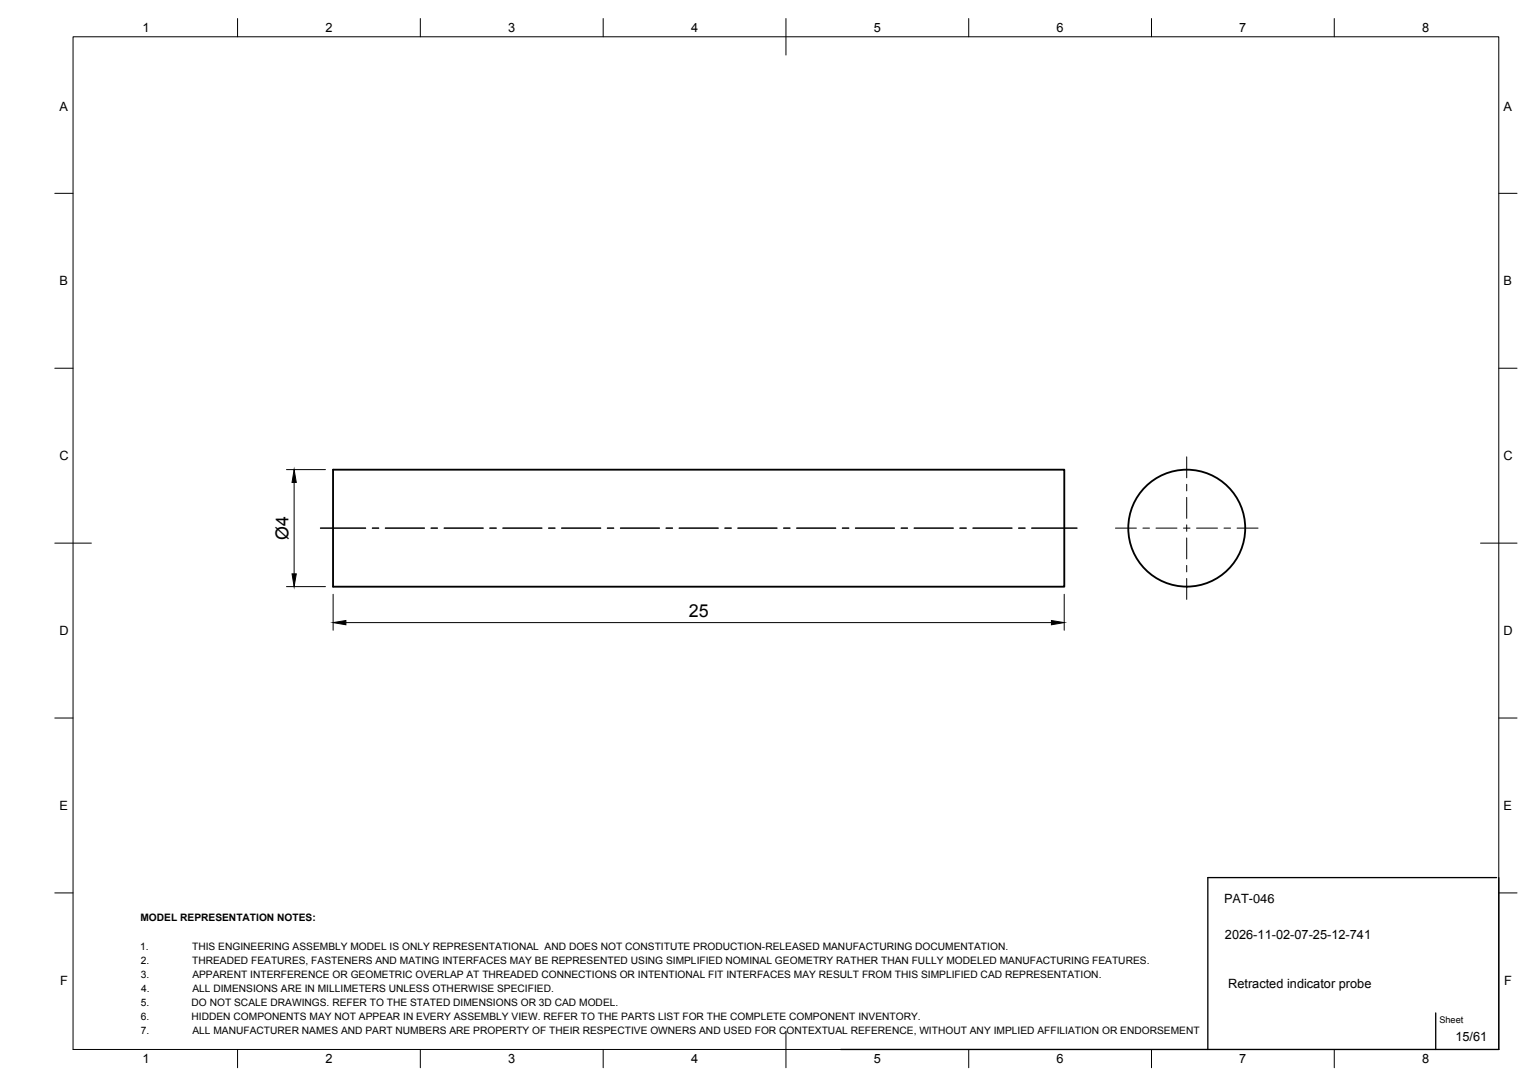
ISO-10303-21;
HEADER;
/* Generated by software containing ST-Developer
 * from STEP Tools, Inc. (www.steptools.com) 
 */

FILE_DESCRIPTION(
/* description */ ('Gear mesh backlash fixture'),
/* implementation_level */ '2;1');

FILE_NAME(
/* name */ 'Retracted indicator probe.step',
/* time_stamp */ '2026-10-28T03:26:00-07:00',
/* author */ (''),
/* organization */ (''),
/* preprocessor_version */ 'ST-DEVELOPER v20.2',
/* originating_system */ 'Autodesk Translation Framework v15.17.0.0',
/* authorisation */ '');

FILE_SCHEMA (('AUTOMOTIVE_DESIGN { 1 0 10303 214 3 1 1 }'));
ENDSEC;

DATA;
#10=MECHANICAL_DESIGN_GEOMETRIC_PRESENTATION_REPRESENTATION('',(#1026),#57900);
#926=SHAPE_REPRESENTATION_RELATIONSHIP('SRR','None',#58121,#976);
#976=ADVANCED_BREP_SHAPE_REPRESENTATION('',(#1091),#57854);
#1026=STYLED_ITEM('',(#58458),#1091);
#1091=MANIFOLD_SOLID_BREP('Body1',#13586);
#1393=PLANE('',#14451);
#1394=PLANE('',#14452);
#1811=FACE_OUTER_BOUND('',#2638,.T.);
#1812=FACE_OUTER_BOUND('',#2639,.T.);
#1813=FACE_OUTER_BOUND('',#2640,.T.);
#2638=EDGE_LOOP('',(#9421,#9422,#9423,#9424));
#2639=EDGE_LOOP('',(#9425));
#2640=EDGE_LOOP('',(#9426));
#3552=LINE('',#19909,#4441);
#4441=VECTOR('',#16229,0.2);
#5312=CIRCLE('',#14449,0.2);
#5313=CIRCLE('',#14450,0.2);
#5957=VERTEX_POINT('',#19906);
#5958=VERTEX_POINT('',#19908);
#7297=EDGE_CURVE('',#5957,#5957,#5312,.T.);
#7298=EDGE_CURVE('',#5957,#5958,#3552,.T.);
#7299=EDGE_CURVE('',#5958,#5958,#5313,.T.);
#9421=ORIENTED_EDGE('',*,*,#7297,.F.);
#9422=ORIENTED_EDGE('',*,*,#7298,.T.);
#9423=ORIENTED_EDGE('',*,*,#7299,.T.);
#9424=ORIENTED_EDGE('',*,*,#7298,.F.);
#9425=ORIENTED_EDGE('',*,*,#7297,.T.);
#9426=ORIENTED_EDGE('',*,*,#7299,.F.);
#12639=CYLINDRICAL_SURFACE('',#14448,0.2);
#12928=ADVANCED_FACE('',(#1811),#12639,.T.);
#12929=ADVANCED_FACE('',(#1812),#1393,.T.);
#12930=ADVANCED_FACE('',(#1813),#1394,.F.);
#13586=CLOSED_SHELL('',(#12928,#12929,#12930));
#14447=AXIS2_PLACEMENT_3D('',#19904,#16223,#16224);
#14448=AXIS2_PLACEMENT_3D('',#19905,#16225,#16226);
#14449=AXIS2_PLACEMENT_3D('',#19907,#16227,#16228);
#14450=AXIS2_PLACEMENT_3D('',#19910,#16230,#16231);
#14451=AXIS2_PLACEMENT_3D('',#19911,#16232,#16233);
#14452=AXIS2_PLACEMENT_3D('',#19912,#16234,#16235);
#16223=DIRECTION('axis',(0.,0.,1.));
#16224=DIRECTION('refdir',(1.,0.,0.));
#16225=DIRECTION('center_axis',(0.,1.,0.));
#16226=DIRECTION('ref_axis',(1.,0.,0.));
#16227=DIRECTION('center_axis',(0.,1.,0.));
#16228=DIRECTION('ref_axis',(1.,0.,0.));
#16229=DIRECTION('',(0.,-1.,0.));
#16230=DIRECTION('center_axis',(0.,1.,0.));
#16231=DIRECTION('ref_axis',(1.,0.,0.));
#16232=DIRECTION('center_axis',(0.,1.,0.));
#16233=DIRECTION('ref_axis',(1.,0.,0.));
#16234=DIRECTION('center_axis',(0.,1.,0.));
#16235=DIRECTION('ref_axis',(1.,0.,0.));
#19904=CARTESIAN_POINT('',(0.,0.,0.));
#19905=CARTESIAN_POINT('Origin',(6.,4.5,12.));
#19906=CARTESIAN_POINT('',(5.8,7.,12.));
#19907=CARTESIAN_POINT('Origin',(6.,7.,12.));
#19908=CARTESIAN_POINT('',(5.8,4.5,12.));
#19909=CARTESIAN_POINT('',(5.8,4.5,12.));
#19910=CARTESIAN_POINT('Origin',(6.,4.5,12.));
#19911=CARTESIAN_POINT('Origin',(6.,7.,12.));
#19912=CARTESIAN_POINT('Origin',(6.,4.5,12.));
#57795=UNCERTAINTY_MEASURE_WITH_UNIT(LENGTH_MEASURE(0.001),#57901,
'DISTANCE_ACCURACY_VALUE',
'Maximum model space distance between geometric entities at asserted c
onnectivities');
#57841=UNCERTAINTY_MEASURE_WITH_UNIT(LENGTH_MEASURE(0.001),#57901,
'DISTANCE_ACCURACY_VALUE',
'Maximum model space distance between geometric entities at asserted c
onnectivities');
#57854=(
GEOMETRIC_REPRESENTATION_CONTEXT(3)
GLOBAL_UNCERTAINTY_ASSIGNED_CONTEXT((#57795))
GLOBAL_UNIT_ASSIGNED_CONTEXT((#57901,#57903,#57904))
REPRESENTATION_CONTEXT('','3D')
);
#57900=(
GEOMETRIC_REPRESENTATION_CONTEXT(3)
GLOBAL_UNCERTAINTY_ASSIGNED_CONTEXT((#57841))
GLOBAL_UNIT_ASSIGNED_CONTEXT((#57901,#57903,#57904))
REPRESENTATION_CONTEXT('','3D')
);
#57901=(
LENGTH_UNIT()
NAMED_UNIT(*)
SI_UNIT(.CENTI.,.METRE.)
);
#57903=(
NAMED_UNIT(*)
PLANE_ANGLE_UNIT()
SI_UNIT($,.RADIAN.)
);
#57904=(
NAMED_UNIT(*)
SI_UNIT($,.STERADIAN.)
SOLID_ANGLE_UNIT()
);
#57917=SHAPE_DEFINITION_REPRESENTATION(#57975,#58121);
#57975=PRODUCT_DEFINITION_SHAPE('',$,#58180);
#58121=SHAPE_REPRESENTATION('',(#14447),#57854);
#58167=PRODUCT_DEFINITION_CONTEXT('part definition',#58343,'design');
#58180=PRODUCT_DEFINITION('Retracted indicator probe',
'Retracted indicator probe',#58238,#58167);
#58238=PRODUCT_DEFINITION_FORMATION('',$,#58357);
#58343=APPLICATION_CONTEXT(
'Core Data for Automotive Mechanical Design Process');
#58344=PRODUCT_CONTEXT('part definition',#58343,'mechanical');
#58357=PRODUCT('Retracted indicator probe','Retracted indicator probe',
'Retracted indicator probe',(#58344));
#58452=COLOUR_RGB('Sky Blue',0.24,0.69,0.87);
#58453=FILL_AREA_STYLE_COLOUR('',#58452);
#58454=FILL_AREA_STYLE('',(#58453));
#58455=SURFACE_STYLE_FILL_AREA(#58454);
#58456=SURFACE_SIDE_STYLE('',(#58455));
#58457=SURFACE_STYLE_USAGE(.BOTH.,#58456);
#58458=PRESENTATION_STYLE_ASSIGNMENT((#58457));
ENDSEC;
END-ISO-10303-21;
